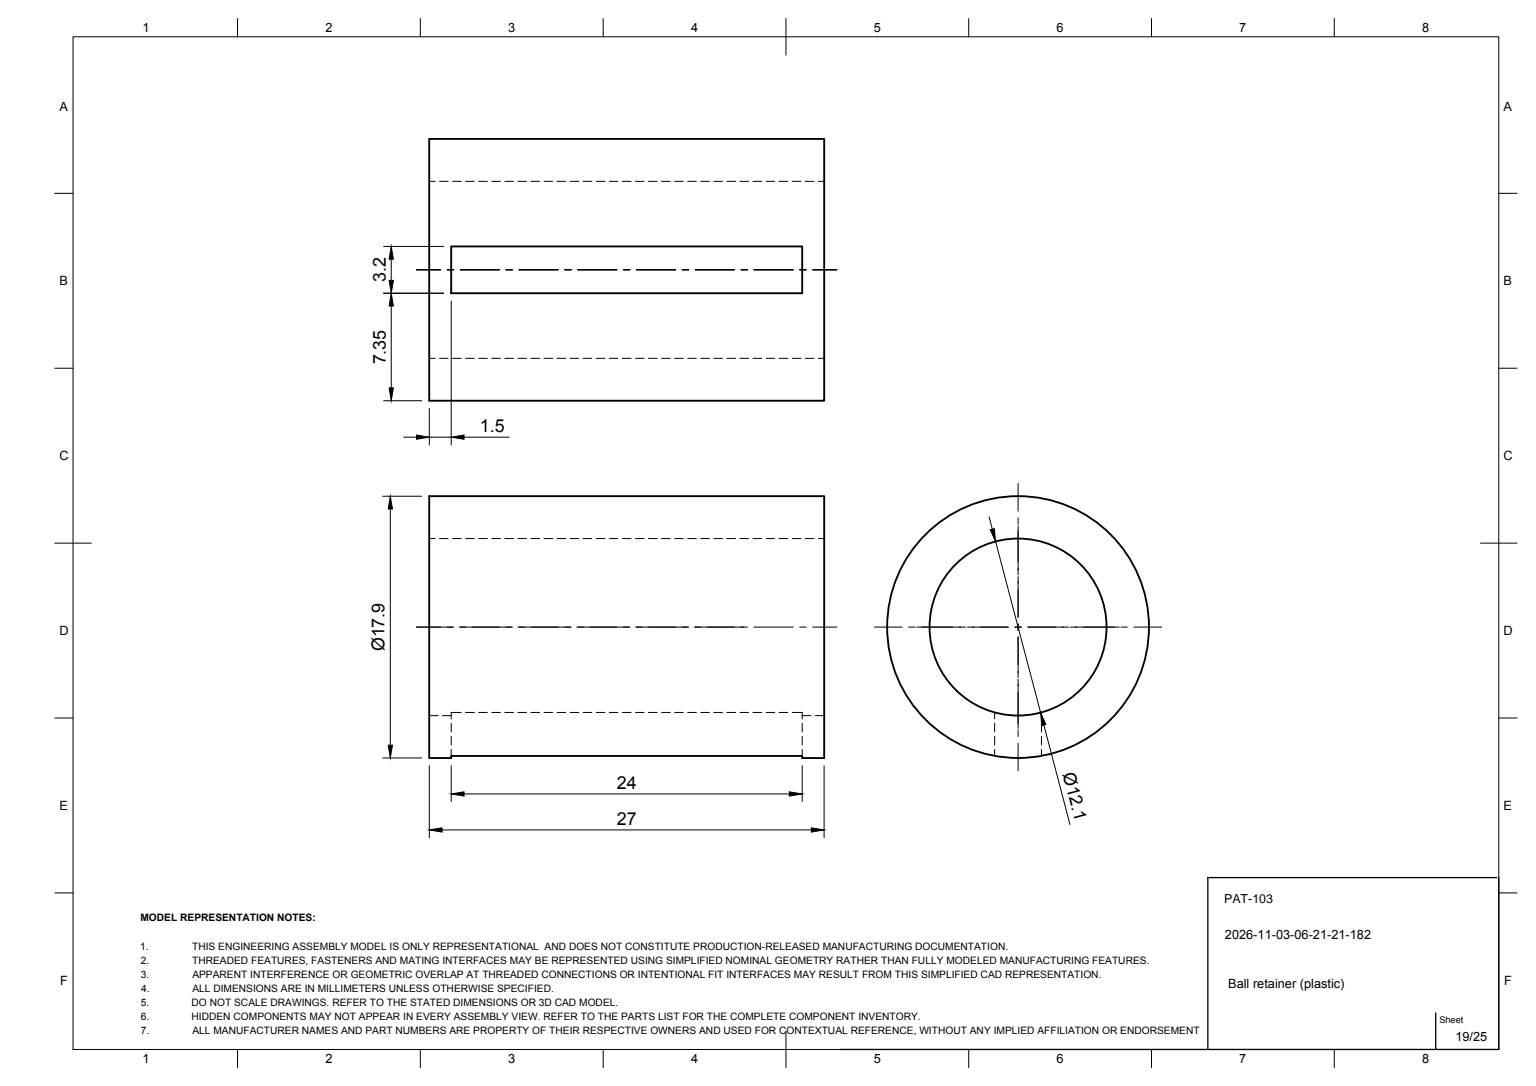
ISO-10303-21;
HEADER;
/* Generated by software containing ST-Developer
 * from STEP Tools, Inc. (www.steptools.com) 
 */

FILE_DESCRIPTION(
/* description */ ('Telescoping shaft support with lock collar'),
/* implementation_level */ '2;1');

FILE_NAME(
/* name */ 'Ball retainer (plastic).step',
/* time_stamp */ '2026-10-27T10:48:51-07:00',
/* author */ (''),
/* organization */ (''),
/* preprocessor_version */ 'ST-DEVELOPER v20.2',
/* originating_system */ 'Autodesk Translation Framework v15.17.0.0',
/* authorisation */ '');

FILE_SCHEMA (('AUTOMOTIVE_DESIGN { 1 0 10303 214 3 1 1 }'));
ENDSEC;

DATA;
#10=MECHANICAL_DESIGN_GEOMETRIC_PRESENTATION_REPRESENTATION('',(#254),#7349);
#214=SHAPE_REPRESENTATION_RELATIONSHIP('SRR','None',#7457,#234);
#234=ADVANCED_BREP_SHAPE_REPRESENTATION('',(#273),#7341);
#254=STYLED_ITEM('',(#7620),#273);
#273=MANIFOLD_SOLID_BREP('Body1',#3978);
#345=FACE_BOUND('',#954,.T.);
#346=FACE_BOUND('',#956,.T.);
#347=FACE_BOUND('',#958,.T.);
#348=FACE_BOUND('',#960,.T.);
#455=PLANE('',#4553);
#456=PLANE('',#4556);
#457=PLANE('',#4557);
#458=PLANE('',#4560);
#459=PLANE('',#4561);
#460=PLANE('',#4566);
#657=FACE_OUTER_BOUND('',#949,.T.);
#658=FACE_OUTER_BOUND('',#950,.T.);
#659=FACE_OUTER_BOUND('',#951,.T.);
#660=FACE_OUTER_BOUND('',#952,.T.);
#661=FACE_OUTER_BOUND('',#953,.T.);
#662=FACE_OUTER_BOUND('',#955,.T.);
#663=FACE_OUTER_BOUND('',#957,.T.);
#664=FACE_OUTER_BOUND('',#959,.T.);
#949=EDGE_LOOP('',(#3392,#3393,#3394,#3395));
#950=EDGE_LOOP('',(#3396,#3397,#3398,#3399));
#951=EDGE_LOOP('',(#3400,#3401,#3402,#3403));
#952=EDGE_LOOP('',(#3404,#3405,#3406,#3407));
#953=EDGE_LOOP('',(#3408));
#954=EDGE_LOOP('',(#3409));
#955=EDGE_LOOP('',(#3410,#3411,#3412,#3413));
#956=EDGE_LOOP('',(#3414,#3415,#3416,#3417));
#957=EDGE_LOOP('',(#3418));
#958=EDGE_LOOP('',(#3419));
#959=EDGE_LOOP('',(#3420,#3421,#3422,#3423));
#960=EDGE_LOOP('',(#3424,#3425,#3426,#3427));
#1231=LINE('',#6865,#1511);
#1232=LINE('',#6868,#1512);
#1233=LINE('',#6871,#1513);
#1234=LINE('',#6873,#1514);
#1235=LINE('',#6874,#1515);
#1236=LINE('',#6880,#1516);
#1237=LINE('',#6882,#1517);
#1238=LINE('',#6883,#1518);
#1239=LINE('',#6892,#1519);
#1240=LINE('',#6897,#1520);
#1511=VECTOR('',#5607,1.);
#1512=VECTOR('',#5610,1.);
#1513=VECTOR('',#5613,1.);
#1514=VECTOR('',#5614,1.);
#1515=VECTOR('',#5615,1.);
#1516=VECTOR('',#5622,1.);
#1517=VECTOR('',#5625,1.);
#1518=VECTOR('',#5626,1.);
#1519=VECTOR('',#5637,0.895);
#1520=VECTOR('',#5644,0.605);
#1754=CIRCLE('',#4554,0.895);
#1755=CIRCLE('',#4555,0.605);
#1756=CIRCLE('',#4558,0.895);
#1757=CIRCLE('',#4559,0.605);
#1758=CIRCLE('',#4562,0.895);
#1759=CIRCLE('',#4563,0.605);
#1760=CIRCLE('',#4565,0.895);
#1761=CIRCLE('',#4567,0.605);
#2047=VERTEX_POINT('',#6861);
#2048=VERTEX_POINT('',#6862);
#2049=VERTEX_POINT('',#6864);
#2050=VERTEX_POINT('',#6866);
#2051=VERTEX_POINT('',#6870);
#2052=VERTEX_POINT('',#6872);
#2053=VERTEX_POINT('',#6876);
#2054=VERTEX_POINT('',#6878);
#2055=VERTEX_POINT('',#6885);
#2056=VERTEX_POINT('',#6887);
#2057=VERTEX_POINT('',#6890);
#2058=VERTEX_POINT('',#6894);
#2508=EDGE_CURVE('',#2047,#2048,#1754,.T.);
#2509=EDGE_CURVE('',#2049,#2047,#1231,.T.);
#2510=EDGE_CURVE('',#2050,#2049,#1755,.T.);
#2511=EDGE_CURVE('',#2048,#2050,#1232,.T.);
#2512=EDGE_CURVE('',#2048,#2051,#1233,.T.);
#2513=EDGE_CURVE('',#2052,#2050,#1234,.T.);
#2514=EDGE_CURVE('',#2052,#2051,#1235,.T.);
#2515=EDGE_CURVE('',#2051,#2053,#1756,.T.);
#2516=EDGE_CURVE('',#2054,#2052,#1757,.T.);
#2517=EDGE_CURVE('',#2053,#2054,#1236,.T.);
#2518=EDGE_CURVE('',#2053,#2047,#1237,.T.);
#2519=EDGE_CURVE('',#2049,#2054,#1238,.T.);
#2520=EDGE_CURVE('',#2055,#2055,#1758,.T.);
#2521=EDGE_CURVE('',#2056,#2056,#1759,.T.);
#2522=EDGE_CURVE('',#2057,#2057,#1760,.T.);
#2523=EDGE_CURVE('',#2057,#2055,#1239,.T.);
#2524=EDGE_CURVE('',#2058,#2058,#1761,.T.);
#2525=EDGE_CURVE('',#2058,#2056,#1240,.T.);
#3392=ORIENTED_EDGE('',*,*,#2508,.F.);
#3393=ORIENTED_EDGE('',*,*,#2509,.F.);
#3394=ORIENTED_EDGE('',*,*,#2510,.F.);
#3395=ORIENTED_EDGE('',*,*,#2511,.F.);
#3396=ORIENTED_EDGE('',*,*,#2512,.F.);
#3397=ORIENTED_EDGE('',*,*,#2511,.T.);
#3398=ORIENTED_EDGE('',*,*,#2513,.F.);
#3399=ORIENTED_EDGE('',*,*,#2514,.T.);
#3400=ORIENTED_EDGE('',*,*,#2515,.F.);
#3401=ORIENTED_EDGE('',*,*,#2514,.F.);
#3402=ORIENTED_EDGE('',*,*,#2516,.F.);
#3403=ORIENTED_EDGE('',*,*,#2517,.F.);
#3404=ORIENTED_EDGE('',*,*,#2518,.F.);
#3405=ORIENTED_EDGE('',*,*,#2517,.T.);
#3406=ORIENTED_EDGE('',*,*,#2519,.F.);
#3407=ORIENTED_EDGE('',*,*,#2509,.T.);
#3408=ORIENTED_EDGE('',*,*,#2520,.F.);
#3409=ORIENTED_EDGE('',*,*,#2521,.T.);
#3410=ORIENTED_EDGE('',*,*,#2522,.F.);
#3411=ORIENTED_EDGE('',*,*,#2523,.T.);
#3412=ORIENTED_EDGE('',*,*,#2520,.T.);
#3413=ORIENTED_EDGE('',*,*,#2523,.F.);
#3414=ORIENTED_EDGE('',*,*,#2515,.T.);
#3415=ORIENTED_EDGE('',*,*,#2518,.T.);
#3416=ORIENTED_EDGE('',*,*,#2508,.T.);
#3417=ORIENTED_EDGE('',*,*,#2512,.T.);
#3418=ORIENTED_EDGE('',*,*,#2522,.T.);
#3419=ORIENTED_EDGE('',*,*,#2524,.F.);
#3420=ORIENTED_EDGE('',*,*,#2524,.T.);
#3421=ORIENTED_EDGE('',*,*,#2525,.T.);
#3422=ORIENTED_EDGE('',*,*,#2521,.F.);
#3423=ORIENTED_EDGE('',*,*,#2525,.F.);
#3424=ORIENTED_EDGE('',*,*,#2516,.T.);
#3425=ORIENTED_EDGE('',*,*,#2513,.T.);
#3426=ORIENTED_EDGE('',*,*,#2510,.T.);
#3427=ORIENTED_EDGE('',*,*,#2519,.T.);
#3722=CYLINDRICAL_SURFACE('',#4564,0.895);
#3723=CYLINDRICAL_SURFACE('',#4568,0.605);
#3900=ADVANCED_FACE('',(#657),#455,.F.);
#3901=ADVANCED_FACE('',(#658),#456,.F.);
#3902=ADVANCED_FACE('',(#659),#457,.F.);
#3903=ADVANCED_FACE('',(#660),#458,.F.);
#3904=ADVANCED_FACE('',(#661,#345),#459,.T.);
#3905=ADVANCED_FACE('',(#662,#346),#3722,.T.);
#3906=ADVANCED_FACE('',(#663,#347),#460,.T.);
#3907=ADVANCED_FACE('',(#664,#348),#3723,.F.);
#3978=CLOSED_SHELL('',(#3900,#3901,#3902,#3903,#3904,#3905,#3906,#3907));
#4552=AXIS2_PLACEMENT_3D('',#6859,#5601,#5602);
#4553=AXIS2_PLACEMENT_3D('',#6860,#5603,#5604);
#4554=AXIS2_PLACEMENT_3D('',#6863,#5605,#5606);
#4555=AXIS2_PLACEMENT_3D('',#6867,#5608,#5609);
#4556=AXIS2_PLACEMENT_3D('',#6869,#5611,#5612);
#4557=AXIS2_PLACEMENT_3D('',#6875,#5616,#5617);
#4558=AXIS2_PLACEMENT_3D('',#6877,#5618,#5619);
#4559=AXIS2_PLACEMENT_3D('',#6879,#5620,#5621);
#4560=AXIS2_PLACEMENT_3D('',#6881,#5623,#5624);
#4561=AXIS2_PLACEMENT_3D('',#6884,#5627,#5628);
#4562=AXIS2_PLACEMENT_3D('',#6886,#5629,#5630);
#4563=AXIS2_PLACEMENT_3D('',#6888,#5631,#5632);
#4564=AXIS2_PLACEMENT_3D('',#6889,#5633,#5634);
#4565=AXIS2_PLACEMENT_3D('',#6891,#5635,#5636);
#4566=AXIS2_PLACEMENT_3D('',#6893,#5638,#5639);
#4567=AXIS2_PLACEMENT_3D('',#6895,#5640,#5641);
#4568=AXIS2_PLACEMENT_3D('',#6896,#5642,#5643);
#5601=DIRECTION('axis',(0.,0.,1.));
#5602=DIRECTION('refdir',(1.,0.,0.));
#5603=DIRECTION('center_axis',(0.,1.,0.));
#5604=DIRECTION('ref_axis',(0.,0.,1.));
#5605=DIRECTION('center_axis',(0.,1.,0.));
#5606=DIRECTION('ref_axis',(1.,0.,0.));
#5607=DIRECTION('',(1.,0.,0.));
#5608=DIRECTION('center_axis',(0.,-1.,0.));
#5609=DIRECTION('ref_axis',(1.,0.,0.));
#5610=DIRECTION('',(-1.,0.,0.));
#5611=DIRECTION('center_axis',(0.,0.,-1.));
#5612=DIRECTION('ref_axis',(-1.,0.,0.));
#5613=DIRECTION('',(0.,-1.,0.));
#5614=DIRECTION('',(0.,1.,0.));
#5615=DIRECTION('',(1.,0.,0.));
#5616=DIRECTION('center_axis',(0.,-1.,0.));
#5617=DIRECTION('ref_axis',(0.,0.,-1.));
#5618=DIRECTION('center_axis',(0.,-1.,0.));
#5619=DIRECTION('ref_axis',(1.,0.,0.));
#5620=DIRECTION('center_axis',(0.,1.,0.));
#5621=DIRECTION('ref_axis',(1.,0.,0.));
#5622=DIRECTION('',(-1.,0.,0.));
#5623=DIRECTION('center_axis',(0.,0.,1.));
#5624=DIRECTION('ref_axis',(1.,0.,0.));
#5625=DIRECTION('',(0.,1.,0.));
#5626=DIRECTION('',(0.,-1.,0.));
#5627=DIRECTION('center_axis',(0.,1.,0.));
#5628=DIRECTION('ref_axis',(0.,0.,1.));
#5629=DIRECTION('center_axis',(0.,-1.,0.));
#5630=DIRECTION('ref_axis',(1.,0.,0.));
#5631=DIRECTION('center_axis',(0.,-1.,0.));
#5632=DIRECTION('ref_axis',(1.,0.,0.));
#5633=DIRECTION('center_axis',(0.,-1.,0.));
#5634=DIRECTION('ref_axis',(1.,0.,0.));
#5635=DIRECTION('center_axis',(0.,-1.,0.));
#5636=DIRECTION('ref_axis',(1.,0.,0.));
#5637=DIRECTION('',(0.,1.,0.));
#5638=DIRECTION('center_axis',(0.,-1.,0.));
#5639=DIRECTION('ref_axis',(0.,0.,-1.));
#5640=DIRECTION('center_axis',(0.,-1.,0.));
#5641=DIRECTION('ref_axis',(1.,0.,0.));
#5642=DIRECTION('center_axis',(0.,-1.,0.));
#5643=DIRECTION('ref_axis',(1.,0.,0.));
#5644=DIRECTION('',(0.,1.,0.));
#6859=CARTESIAN_POINT('',(0.,0.,0.));
#6860=CARTESIAN_POINT('Origin',(0.75,1.2,0.));
#6861=CARTESIAN_POINT('',(0.880582193778639,1.2,0.16));
#6862=CARTESIAN_POINT('',(0.880582193778639,1.2,-0.16));
#6863=CARTESIAN_POINT('Origin',(0.,1.2,0.));
#6864=CARTESIAN_POINT('',(0.583459510163302,1.2,0.16));
#6865=CARTESIAN_POINT('',(0.57,1.2,0.16));
#6866=CARTESIAN_POINT('',(0.583459510163302,1.2,-0.16));
#6867=CARTESIAN_POINT('Origin',(0.,1.2,0.));
#6868=CARTESIAN_POINT('',(0.93,1.2,-0.16));
#6869=CARTESIAN_POINT('Origin',(0.93,0.,-0.16));
#6870=CARTESIAN_POINT('',(0.880582193778639,-1.2,-0.16));
#6871=CARTESIAN_POINT('',(0.880582193778639,0.,-0.16));
#6872=CARTESIAN_POINT('',(0.583459510163302,-1.2,-0.16));
#6873=CARTESIAN_POINT('',(0.583459510163302,0.,-0.16));
#6874=CARTESIAN_POINT('',(0.93,-1.2,-0.16));
#6875=CARTESIAN_POINT('Origin',(0.75,-1.2,0.));
#6876=CARTESIAN_POINT('',(0.880582193778639,-1.2,0.16));
#6877=CARTESIAN_POINT('Origin',(0.,-1.2,0.));
#6878=CARTESIAN_POINT('',(0.583459510163302,-1.2,0.16));
#6879=CARTESIAN_POINT('Origin',(0.,-1.2,0.));
#6880=CARTESIAN_POINT('',(0.57,-1.2,0.16));
#6881=CARTESIAN_POINT('Origin',(0.57,0.,0.16));
#6882=CARTESIAN_POINT('',(0.880582193778639,0.,0.16));
#6883=CARTESIAN_POINT('',(0.583459510163302,0.,0.16));
#6884=CARTESIAN_POINT('Origin',(0.895,1.35,0.));
#6885=CARTESIAN_POINT('',(-0.895,1.35,-1.09605888523688E-16));
#6886=CARTESIAN_POINT('Origin',(0.,1.35,0.));
#6887=CARTESIAN_POINT('',(-0.605,1.35,-7.40911313484149E-17));
#6888=CARTESIAN_POINT('Origin',(0.,1.35,0.));
#6889=CARTESIAN_POINT('Origin',(0.,0.,0.));
#6890=CARTESIAN_POINT('',(-0.895,-1.35,-1.09605888523688E-16));
#6891=CARTESIAN_POINT('Origin',(0.,-1.35,0.));
#6892=CARTESIAN_POINT('',(-0.895,0.,-1.09605888523688E-16));
#6893=CARTESIAN_POINT('Origin',(0.605,-1.35,0.));
#6894=CARTESIAN_POINT('',(-0.605,-1.35,-7.40911313484149E-17));
#6895=CARTESIAN_POINT('Origin',(0.,-1.35,0.));
#6896=CARTESIAN_POINT('Origin',(0.,0.,0.));
#6897=CARTESIAN_POINT('',(-0.605,0.,-7.40911313484149E-17));
#7316=UNCERTAINTY_MEASURE_WITH_UNIT(LENGTH_MEASURE(0.001),#7350,
'DISTANCE_ACCURACY_VALUE',
'Maximum model space distance between geometric entities at asserted c
onnectivities');
#7324=UNCERTAINTY_MEASURE_WITH_UNIT(LENGTH_MEASURE(0.001),#7350,
'DISTANCE_ACCURACY_VALUE',
'Maximum model space distance between geometric entities at asserted c
onnectivities');
#7341=(
GEOMETRIC_REPRESENTATION_CONTEXT(3)
GLOBAL_UNCERTAINTY_ASSIGNED_CONTEXT((#7316))
GLOBAL_UNIT_ASSIGNED_CONTEXT((#7350,#7352,#7353))
REPRESENTATION_CONTEXT('','3D')
);
#7349=(
GEOMETRIC_REPRESENTATION_CONTEXT(3)
GLOBAL_UNCERTAINTY_ASSIGNED_CONTEXT((#7324))
GLOBAL_UNIT_ASSIGNED_CONTEXT((#7350,#7352,#7353))
REPRESENTATION_CONTEXT('','3D')
);
#7350=(
LENGTH_UNIT()
NAMED_UNIT(*)
SI_UNIT(.CENTI.,.METRE.)
);
#7352=(
NAMED_UNIT(*)
PLANE_ANGLE_UNIT()
SI_UNIT($,.RADIAN.)
);
#7353=(
NAMED_UNIT(*)
SI_UNIT($,.STERADIAN.)
SOLID_ANGLE_UNIT()
);
#7370=SHAPE_DEFINITION_REPRESENTATION(#7394,#7457);
#7394=PRODUCT_DEFINITION_SHAPE('',$,#7482);
#7457=SHAPE_REPRESENTATION('',(#4552),#7341);
#7465=PRODUCT_DEFINITION_CONTEXT('part definition',#7539,'design');
#7482=PRODUCT_DEFINITION('Ball retainer (plastic)',
'Ball retainer (plastic)',#7506,#7465);
#7506=PRODUCT_DEFINITION_FORMATION('',$,#7557);
#7539=APPLICATION_CONTEXT(
'Core Data for Automotive Mechanical Design Process');
#7540=PRODUCT_CONTEXT('part definition',#7539,'mechanical');
#7557=PRODUCT('Ball retainer (plastic)','Ball retainer (plastic)',
'Ball retainer (plastic)',(#7540));
#7614=COLOUR_RGB('Sky Blue',0.24,0.69,0.87);
#7615=FILL_AREA_STYLE_COLOUR('',#7614);
#7616=FILL_AREA_STYLE('',(#7615));
#7617=SURFACE_STYLE_FILL_AREA(#7616);
#7618=SURFACE_SIDE_STYLE('',(#7617));
#7619=SURFACE_STYLE_USAGE(.BOTH.,#7618);
#7620=PRESENTATION_STYLE_ASSIGNMENT((#7619));
ENDSEC;
END-ISO-10303-21;
